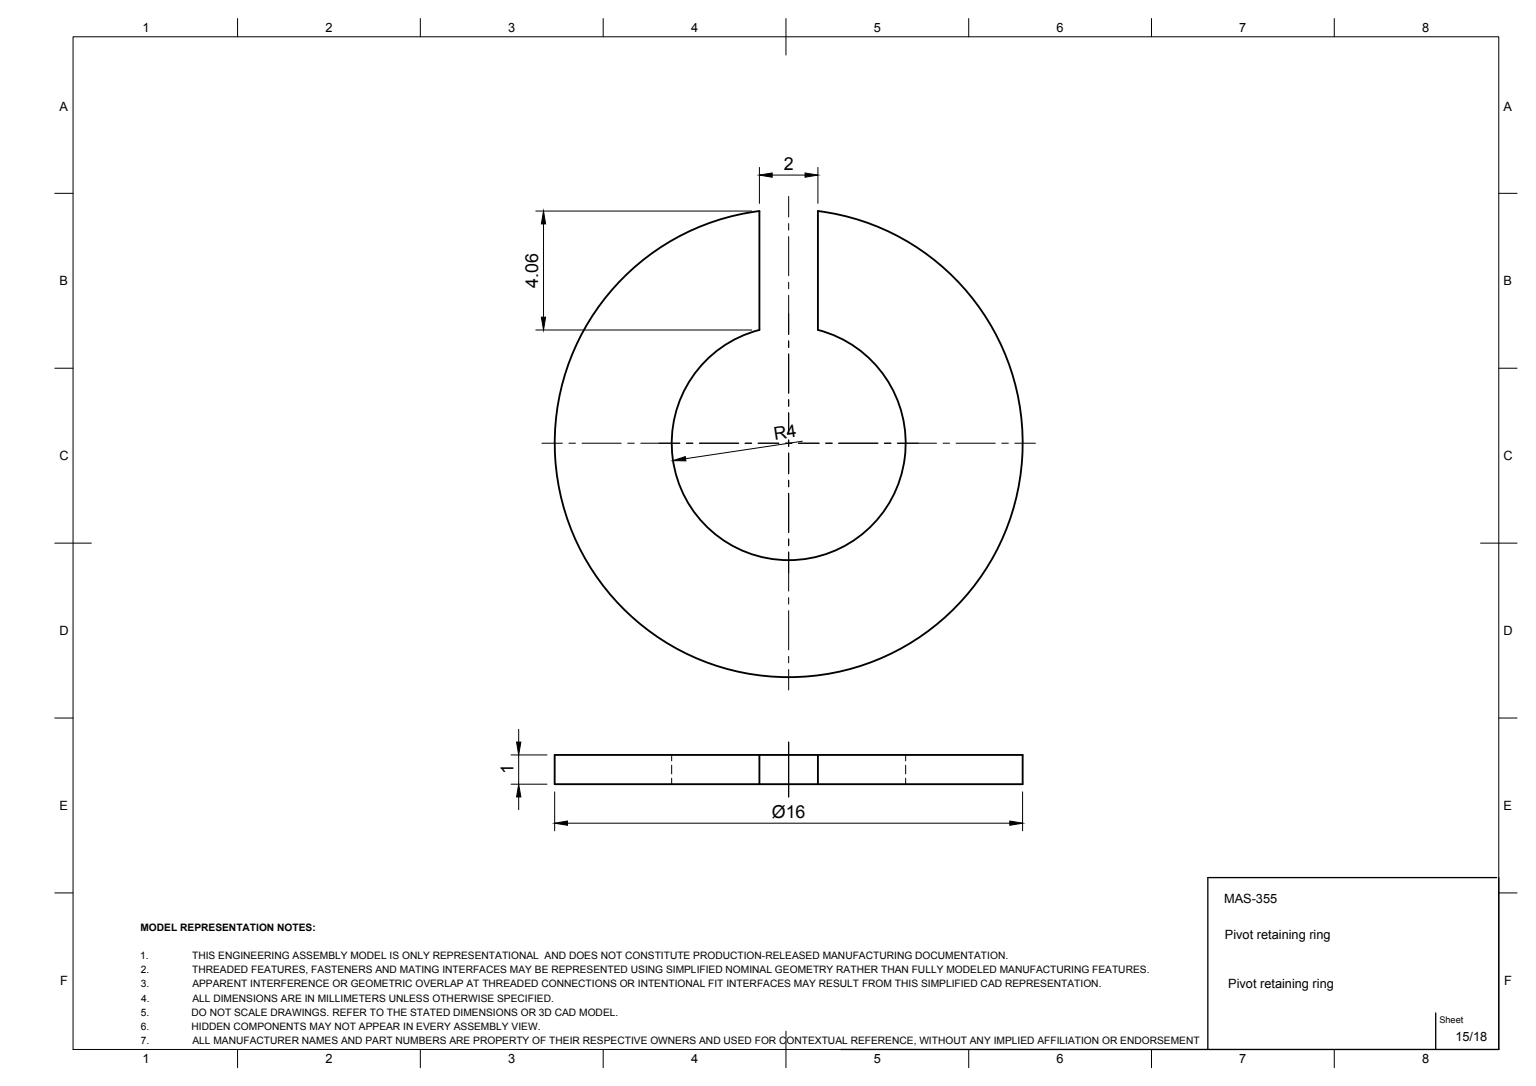
ISO-10303-21;
HEADER;
/* Generated by software containing ST-Developer
 * from STEP Tools, Inc. (www.steptools.com) 
 */

FILE_DESCRIPTION(
/* description */ ('Independent two-stage fixed-ring planetary gearbox,24/24/72 teeth,mod
ule2,20deg involutes,three planets per stage,4:1 x4:1=16:1. Native cut
-space/fillet/pattern tooth profiles derived from reusable gear blanks
; shared sun/planet/ring/carrier parts across both stages. Captured br
onze-journal input/carriers, headed retained planet pins, keyed inters
tage drive and modular keyed output interface. Native ideal gear links
; no torque, precision grade, production backlash/fits, lubrication, s
peed or life rating.'),
/* implementation_level */ '2;1');

FILE_NAME(
/* name */ 'Pivot retaining ring.step',
/* time_stamp */ '2026-11-08T19:10:00-08:00',
/* author */ (''),
/* organization */ (''),
/* preprocessor_version */ 'ST-DEVELOPER v20.2',
/* originating_system */ 'Autodesk Translation Framework v15.17.0.0',
/* authorisation */ '');

FILE_SCHEMA (('AUTOMOTIVE_DESIGN { 1 0 10303 214 3 1 1 }'));
ENDSEC;

DATA;
#10=MECHANICAL_DESIGN_GEOMETRIC_PRESENTATION_REPRESENTATION('',(#1175),#259224);
#1135=SHAPE_REPRESENTATION_RELATIONSHIP('SRR','None',#259382,#1155);
#1155=ADVANCED_BREP_SHAPE_REPRESENTATION('',(#1195),#259216);
#1175=STYLED_ITEM('',(#259489),#1195);
#1195=MANIFOLD_SOLID_BREP('Body1',#25162);
#1668=PLANE('',#27111);
#1669=PLANE('',#27112);
#1670=PLANE('',#27113);
#1671=PLANE('',#27120);
#2956=FACE_OUTER_BOUND('',#4409,.T.);
#2957=FACE_OUTER_BOUND('',#4410,.T.);
#2958=FACE_OUTER_BOUND('',#4411,.T.);
#2959=FACE_OUTER_BOUND('',#4412,.T.);
#2960=FACE_OUTER_BOUND('',#4413,.T.);
#2961=FACE_OUTER_BOUND('',#4414,.T.);
#4409=EDGE_LOOP('',(#22658,#22659,#22660,#22661));
#4410=EDGE_LOOP('',(#22662,#22663,#22664,#22665));
#4411=EDGE_LOOP('',(#22666,#22667,#22668,#22669));
#4412=EDGE_LOOP('',(#22670,#22671,#22672,#22673));
#4413=EDGE_LOOP('',(#22674,#22675,#22676,#22677));
#4414=EDGE_LOOP('',(#22678,#22679,#22680,#22681));
#5353=CIRCLE('',#27114,8.);
#5354=CIRCLE('',#27115,4.);
#5355=CIRCLE('',#27117,4.);
#5356=CIRCLE('',#27119,8.);
#7762=LINE('',#255977,#8947);
#7763=LINE('',#255979,#8948);
#7764=LINE('',#255981,#8949);
#7765=LINE('',#255982,#8950);
#7766=LINE('',#255986,#8951);
#7767=LINE('',#255988,#8952);
#7768=LINE('',#255990,#8953);
#7769=LINE('',#255991,#8954);
#8947=VECTOR('',#31871,10.);
#8948=VECTOR('',#31872,10.);
#8949=VECTOR('',#31873,10.);
#8950=VECTOR('',#31874,10.);
#8951=VECTOR('',#31877,10.);
#8952=VECTOR('',#31878,10.);
#8953=VECTOR('',#31879,10.);
#8954=VECTOR('',#31880,10.);
#11457=VERTEX_POINT('',#255975);
#11458=VERTEX_POINT('',#255976);
#11459=VERTEX_POINT('',#255978);
#11460=VERTEX_POINT('',#255980);
#11461=VERTEX_POINT('',#255984);
#11462=VERTEX_POINT('',#255985);
#11463=VERTEX_POINT('',#255987);
#11464=VERTEX_POINT('',#255989);
#15214=EDGE_CURVE('',#11457,#11458,#7762,.T.);
#15215=EDGE_CURVE('',#11459,#11457,#7763,.T.);
#15216=EDGE_CURVE('',#11460,#11459,#7764,.T.);
#15217=EDGE_CURVE('',#11458,#11460,#7765,.T.);
#15218=EDGE_CURVE('',#11461,#11462,#7766,.T.);
#15219=EDGE_CURVE('',#11463,#11461,#7767,.T.);
#15220=EDGE_CURVE('',#11464,#11463,#7768,.T.);
#15221=EDGE_CURVE('',#11462,#11464,#7769,.T.);
#15222=EDGE_CURVE('',#11459,#11464,#5353,.T.);
#15223=EDGE_CURVE('',#11462,#11457,#5354,.T.);
#15224=EDGE_CURVE('',#11461,#11458,#5355,.T.);
#15225=EDGE_CURVE('',#11460,#11463,#5356,.T.);
#22658=ORIENTED_EDGE('',*,*,#15214,.F.);
#22659=ORIENTED_EDGE('',*,*,#15215,.F.);
#22660=ORIENTED_EDGE('',*,*,#15216,.F.);
#22661=ORIENTED_EDGE('',*,*,#15217,.F.);
#22662=ORIENTED_EDGE('',*,*,#15218,.F.);
#22663=ORIENTED_EDGE('',*,*,#15219,.F.);
#22664=ORIENTED_EDGE('',*,*,#15220,.F.);
#22665=ORIENTED_EDGE('',*,*,#15221,.F.);
#22666=ORIENTED_EDGE('',*,*,#15221,.T.);
#22667=ORIENTED_EDGE('',*,*,#15222,.F.);
#22668=ORIENTED_EDGE('',*,*,#15215,.T.);
#22669=ORIENTED_EDGE('',*,*,#15223,.F.);
#22670=ORIENTED_EDGE('',*,*,#15218,.T.);
#22671=ORIENTED_EDGE('',*,*,#15223,.T.);
#22672=ORIENTED_EDGE('',*,*,#15214,.T.);
#22673=ORIENTED_EDGE('',*,*,#15224,.F.);
#22674=ORIENTED_EDGE('',*,*,#15220,.T.);
#22675=ORIENTED_EDGE('',*,*,#15225,.F.);
#22676=ORIENTED_EDGE('',*,*,#15216,.T.);
#22677=ORIENTED_EDGE('',*,*,#15222,.T.);
#22678=ORIENTED_EDGE('',*,*,#15219,.T.);
#22679=ORIENTED_EDGE('',*,*,#15224,.T.);
#22680=ORIENTED_EDGE('',*,*,#15217,.T.);
#22681=ORIENTED_EDGE('',*,*,#15225,.T.);
#23748=CYLINDRICAL_SURFACE('',#27116,4.);
#23749=CYLINDRICAL_SURFACE('',#27118,8.);
#25062=ADVANCED_FACE('',(#2956),#1668,.F.);
#25063=ADVANCED_FACE('',(#2957),#1669,.F.);
#25064=ADVANCED_FACE('',(#2958),#1670,.F.);
#25065=ADVANCED_FACE('',(#2959),#23748,.F.);
#25066=ADVANCED_FACE('',(#2960),#23749,.T.);
#25067=ADVANCED_FACE('',(#2961),#1671,.T.);
#25162=CLOSED_SHELL('',(#25062,#25063,#25064,#25065,#25066,#25067));
#27110=AXIS2_PLACEMENT_3D('',#255973,#31867,#31868);
#27111=AXIS2_PLACEMENT_3D('',#255974,#31869,#31870);
#27112=AXIS2_PLACEMENT_3D('',#255983,#31875,#31876);
#27113=AXIS2_PLACEMENT_3D('',#255992,#31881,#31882);
#27114=AXIS2_PLACEMENT_3D('',#255993,#31883,#31884);
#27115=AXIS2_PLACEMENT_3D('',#255994,#31885,#31886);
#27116=AXIS2_PLACEMENT_3D('',#255995,#31887,#31888);
#27117=AXIS2_PLACEMENT_3D('',#255996,#31889,#31890);
#27118=AXIS2_PLACEMENT_3D('',#255997,#31891,#31892);
#27119=AXIS2_PLACEMENT_3D('',#255998,#31893,#31894);
#27120=AXIS2_PLACEMENT_3D('',#255999,#31895,#31896);
#31867=DIRECTION('axis',(0.,0.,1.));
#31868=DIRECTION('refdir',(1.,0.,0.));
#31869=DIRECTION('center_axis',(-1.,0.,0.));
#31870=DIRECTION('ref_axis',(0.,1.,0.));
#31871=DIRECTION('',(0.,0.,1.));
#31872=DIRECTION('',(0.,-1.,0.));
#31873=DIRECTION('',(0.,0.,-1.));
#31874=DIRECTION('',(0.,1.,0.));
#31875=DIRECTION('center_axis',(1.,0.,0.));
#31876=DIRECTION('ref_axis',(0.,-1.,0.));
#31877=DIRECTION('',(0.,0.,-1.));
#31878=DIRECTION('',(0.,-1.,0.));
#31879=DIRECTION('',(0.,0.,1.));
#31880=DIRECTION('',(0.,1.,0.));
#31881=DIRECTION('center_axis',(0.,0.,1.));
#31882=DIRECTION('ref_axis',(1.,0.,0.));
#31883=DIRECTION('center_axis',(0.,0.,1.));
#31884=DIRECTION('ref_axis',(1.,0.,0.));
#31885=DIRECTION('center_axis',(0.,0.,-1.));
#31886=DIRECTION('ref_axis',(1.,0.,0.));
#31887=DIRECTION('center_axis',(0.,0.,1.));
#31888=DIRECTION('ref_axis',(6.12323399573677E-17,-1.,0.));
#31889=DIRECTION('center_axis',(0.,0.,-1.));
#31890=DIRECTION('ref_axis',(1.,0.,0.));
#31891=DIRECTION('center_axis',(0.,0.,1.));
#31892=DIRECTION('ref_axis',(6.12323399573677E-17,-1.,0.));
#31893=DIRECTION('center_axis',(0.,0.,1.));
#31894=DIRECTION('ref_axis',(1.,0.,0.));
#31895=DIRECTION('center_axis',(0.,0.,1.));
#31896=DIRECTION('ref_axis',(1.,0.,0.));
#255973=CARTESIAN_POINT('',(0.,0.,0.));
#255974=CARTESIAN_POINT('Origin',(-1.,0.,1.));
#255975=CARTESIAN_POINT('',(-1.,3.87298334620742,0.));
#255976=CARTESIAN_POINT('',(-1.,3.87298334620742,1.));
#255977=CARTESIAN_POINT('',(-1.,3.87298334620742,0.));
#255978=CARTESIAN_POINT('',(-1.,7.93725393319377,0.));
#255979=CARTESIAN_POINT('',(-1.,0.,0.));
#255980=CARTESIAN_POINT('',(-1.,7.93725393319377,1.));
#255981=CARTESIAN_POINT('',(-1.,7.93725393319377,0.));
#255982=CARTESIAN_POINT('',(-1.,0.,1.));
#255983=CARTESIAN_POINT('Origin',(1.,16.,1.));
#255984=CARTESIAN_POINT('',(1.,3.87298334620742,1.));
#255985=CARTESIAN_POINT('',(1.,3.87298334620742,0.));
#255986=CARTESIAN_POINT('',(1.,3.87298334620742,0.));
#255987=CARTESIAN_POINT('',(1.,7.93725393319377,1.));
#255988=CARTESIAN_POINT('',(1.,8.,1.));
#255989=CARTESIAN_POINT('',(1.,7.93725393319377,0.));
#255990=CARTESIAN_POINT('',(1.,7.93725393319377,0.));
#255991=CARTESIAN_POINT('',(1.,8.,0.));
#255992=CARTESIAN_POINT('Origin',(0.,0.,0.));
#255993=CARTESIAN_POINT('Origin',(0.,0.,0.));
#255994=CARTESIAN_POINT('Origin',(0.,0.,0.));
#255995=CARTESIAN_POINT('Origin',(0.,0.,0.));
#255996=CARTESIAN_POINT('Origin',(0.,0.,1.));
#255997=CARTESIAN_POINT('Origin',(0.,0.,0.));
#255998=CARTESIAN_POINT('Origin',(0.,0.,1.));
#255999=CARTESIAN_POINT('Origin',(0.,0.,1.));
#259194=UNCERTAINTY_MEASURE_WITH_UNIT(LENGTH_MEASURE(0.01),#259225,
'DISTANCE_ACCURACY_VALUE',
'Maximum model space distance between geometric entities at asserted c
onnectivities');
#259202=UNCERTAINTY_MEASURE_WITH_UNIT(LENGTH_MEASURE(0.01),#259225,
'DISTANCE_ACCURACY_VALUE',
'Maximum model space distance between geometric entities at asserted c
onnectivities');
#259216=(
GEOMETRIC_REPRESENTATION_CONTEXT(3)
GLOBAL_UNCERTAINTY_ASSIGNED_CONTEXT((#259194))
GLOBAL_UNIT_ASSIGNED_CONTEXT((#259225,#259227,#259228))
REPRESENTATION_CONTEXT('','3D')
);
#259224=(
GEOMETRIC_REPRESENTATION_CONTEXT(3)
GLOBAL_UNCERTAINTY_ASSIGNED_CONTEXT((#259202))
GLOBAL_UNIT_ASSIGNED_CONTEXT((#259225,#259227,#259228))
REPRESENTATION_CONTEXT('','3D')
);
#259225=(
LENGTH_UNIT()
NAMED_UNIT(*)
SI_UNIT(.MILLI.,.METRE.)
);
#259227=(
NAMED_UNIT(*)
PLANE_ANGLE_UNIT()
SI_UNIT($,.RADIAN.)
);
#259228=(
NAMED_UNIT(*)
SI_UNIT($,.STERADIAN.)
SOLID_ANGLE_UNIT()
);
#259242=SHAPE_DEFINITION_REPRESENTATION(#259263,#259382);
#259263=PRODUCT_DEFINITION_SHAPE('',$,#259404);
#259382=SHAPE_REPRESENTATION('',(#27110),#259216);
#259390=PRODUCT_DEFINITION_CONTEXT('part definition',#259455,'design');
#259404=PRODUCT_DEFINITION('Pivot retaining ring',
'Pivot retaining ring',#259425,#259390);
#259425=PRODUCT_DEFINITION_FORMATION('',$,#259470);
#259455=APPLICATION_CONTEXT(
'Core Data for Automotive Mechanical Design Process');
#259456=PRODUCT_CONTEXT('part definition',#259455,'mechanical');
#259470=PRODUCT('Pivot retaining ring','Pivot retaining ring',$,(#259456));
#259489=PRESENTATION_STYLE_ASSIGNMENT((#259504));
#259504=SURFACE_STYLE_USAGE(.BOTH.,#259519);
#259519=SURFACE_SIDE_STYLE('',(#259534));
#259534=SURFACE_STYLE_FILL_AREA(#259549);
#259549=FILL_AREA_STYLE('Dark gray',(#259564));
#259564=FILL_AREA_STYLE_COLOUR('Dark gray',#259579);
#259579=COLOUR_RGB('Dark gray',0.250980392156863,0.282352941176471,0.32156862745098);
ENDSEC;
END-ISO-10303-21;
